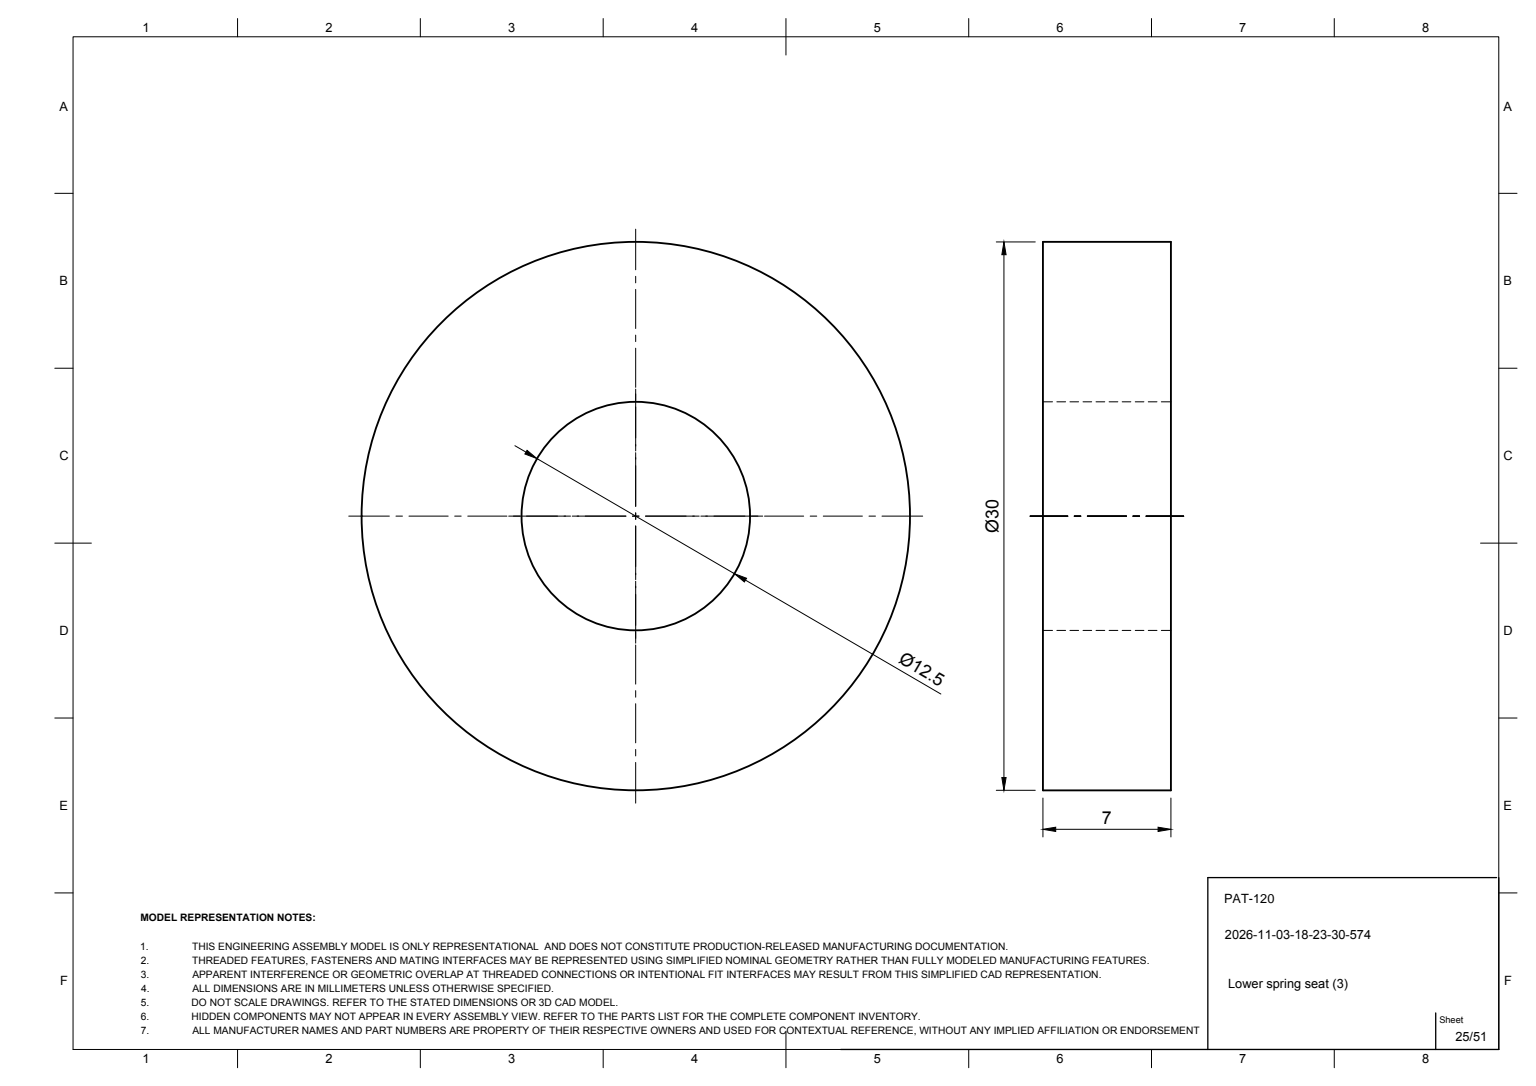
ISO-10303-21;
HEADER;
/* Generated by software containing ST-Developer
 * from STEP Tools, Inc. (www.steptools.com) 
 */

FILE_DESCRIPTION(
/* description */ ('Vibration shaker table dummy'),
/* implementation_level */ '2;1');

FILE_NAME(
/* name */ 'Lower spring seat (3).step',
/* time_stamp */ '2026-10-27T10:55:14-07:00',
/* author */ (''),
/* organization */ (''),
/* preprocessor_version */ 'ST-DEVELOPER v20.2',
/* originating_system */ 'Autodesk Translation Framework v15.17.0.0',
/* authorisation */ '');

FILE_SCHEMA (('AUTOMOTIVE_DESIGN { 1 0 10303 214 3 1 1 }'));
ENDSEC;

DATA;
#10=MECHANICAL_DESIGN_GEOMETRIC_PRESENTATION_REPRESENTATION('',(#706),#22394);
#614=SHAPE_REPRESENTATION_RELATIONSHIP('SRR','None',#22660,#660);
#660=ADVANCED_BREP_SHAPE_REPRESENTATION('',(#752),#22366);
#706=STYLED_ITEM('',(#22961),#752);
#752=MANIFOLD_SOLID_BREP('Body1',#9224);
#917=FACE_BOUND('',#2201,.T.);
#918=FACE_BOUND('',#2203,.T.);
#1188=PLANE('',#10197);
#1189=PLANE('',#10198);
#1558=FACE_OUTER_BOUND('',#2198,.T.);
#1559=FACE_OUTER_BOUND('',#2199,.T.);
#1560=FACE_OUTER_BOUND('',#2200,.T.);
#1561=FACE_OUTER_BOUND('',#2202,.T.);
#2198=EDGE_LOOP('',(#7260,#7261,#7262,#7263));
#2199=EDGE_LOOP('',(#7264,#7265,#7266,#7267));
#2200=EDGE_LOOP('',(#7268));
#2201=EDGE_LOOP('',(#7269));
#2202=EDGE_LOOP('',(#7270));
#2203=EDGE_LOOP('',(#7271));
#2932=LINE('',#19421,#3551);
#2933=LINE('',#19427,#3552);
#3551=VECTOR('',#12126,0.625);
#3552=VECTOR('',#12133,1.5);
#4054=CIRCLE('',#10192,0.625);
#4055=CIRCLE('',#10193,0.625);
#4056=CIRCLE('',#10195,1.5);
#4057=CIRCLE('',#10196,1.5);
#4705=VERTEX_POINT('',#19418);
#4706=VERTEX_POINT('',#19420);
#4707=VERTEX_POINT('',#19424);
#4708=VERTEX_POINT('',#19426);
#5623=EDGE_CURVE('',#4705,#4705,#4054,.T.);
#5624=EDGE_CURVE('',#4705,#4706,#2932,.T.);
#5625=EDGE_CURVE('',#4706,#4706,#4055,.T.);
#5626=EDGE_CURVE('',#4707,#4707,#4056,.T.);
#5627=EDGE_CURVE('',#4707,#4708,#2933,.T.);
#5628=EDGE_CURVE('',#4708,#4708,#4057,.T.);
#7260=ORIENTED_EDGE('',*,*,#5623,.F.);
#7261=ORIENTED_EDGE('',*,*,#5624,.T.);
#7262=ORIENTED_EDGE('',*,*,#5625,.T.);
#7263=ORIENTED_EDGE('',*,*,#5624,.F.);
#7264=ORIENTED_EDGE('',*,*,#5626,.F.);
#7265=ORIENTED_EDGE('',*,*,#5627,.T.);
#7266=ORIENTED_EDGE('',*,*,#5628,.T.);
#7267=ORIENTED_EDGE('',*,*,#5627,.F.);
#7268=ORIENTED_EDGE('',*,*,#5626,.T.);
#7269=ORIENTED_EDGE('',*,*,#5623,.T.);
#7270=ORIENTED_EDGE('',*,*,#5628,.F.);
#7271=ORIENTED_EDGE('',*,*,#5625,.F.);
#8592=CYLINDRICAL_SURFACE('',#10191,0.625);
#8593=CYLINDRICAL_SURFACE('',#10194,1.5);
#8923=ADVANCED_FACE('',(#1558),#8592,.F.);
#8924=ADVANCED_FACE('',(#1559),#8593,.T.);
#8925=ADVANCED_FACE('',(#1560,#917),#1188,.T.);
#8926=ADVANCED_FACE('',(#1561,#918),#1189,.F.);
#9224=CLOSED_SHELL('',(#8923,#8924,#8925,#8926));
#10190=AXIS2_PLACEMENT_3D('',#19416,#12120,#12121);
#10191=AXIS2_PLACEMENT_3D('',#19417,#12122,#12123);
#10192=AXIS2_PLACEMENT_3D('',#19419,#12124,#12125);
#10193=AXIS2_PLACEMENT_3D('',#19422,#12127,#12128);
#10194=AXIS2_PLACEMENT_3D('',#19423,#12129,#12130);
#10195=AXIS2_PLACEMENT_3D('',#19425,#12131,#12132);
#10196=AXIS2_PLACEMENT_3D('',#19428,#12134,#12135);
#10197=AXIS2_PLACEMENT_3D('',#19429,#12136,#12137);
#10198=AXIS2_PLACEMENT_3D('',#19430,#12138,#12139);
#12120=DIRECTION('axis',(0.,0.,1.));
#12121=DIRECTION('refdir',(1.,0.,0.));
#12122=DIRECTION('center_axis',(0.,0.,1.));
#12123=DIRECTION('ref_axis',(1.,0.,0.));
#12124=DIRECTION('center_axis',(0.,0.,-1.));
#12125=DIRECTION('ref_axis',(1.,0.,0.));
#12126=DIRECTION('',(0.,0.,-1.));
#12127=DIRECTION('center_axis',(0.,0.,-1.));
#12128=DIRECTION('ref_axis',(1.,0.,0.));
#12129=DIRECTION('center_axis',(0.,0.,1.));
#12130=DIRECTION('ref_axis',(1.,0.,0.));
#12131=DIRECTION('center_axis',(0.,0.,1.));
#12132=DIRECTION('ref_axis',(1.,0.,0.));
#12133=DIRECTION('',(0.,0.,-1.));
#12134=DIRECTION('center_axis',(0.,0.,1.));
#12135=DIRECTION('ref_axis',(1.,0.,0.));
#12136=DIRECTION('center_axis',(0.,0.,1.));
#12137=DIRECTION('ref_axis',(1.,0.,0.));
#12138=DIRECTION('center_axis',(0.,0.,1.));
#12139=DIRECTION('ref_axis',(1.,0.,0.));
#19416=CARTESIAN_POINT('',(0.,0.,0.));
#19417=CARTESIAN_POINT('Origin',(6.,4.,1.9));
#19418=CARTESIAN_POINT('',(5.375,4.,2.6));
#19419=CARTESIAN_POINT('Origin',(6.,4.,2.6));
#19420=CARTESIAN_POINT('',(5.375,4.,1.9));
#19421=CARTESIAN_POINT('',(5.375,4.,1.9));
#19422=CARTESIAN_POINT('Origin',(6.,4.,1.9));
#19423=CARTESIAN_POINT('Origin',(6.,4.,1.9));
#19424=CARTESIAN_POINT('',(4.5,4.,2.6));
#19425=CARTESIAN_POINT('Origin',(6.,4.,2.6));
#19426=CARTESIAN_POINT('',(4.5,4.,1.9));
#19427=CARTESIAN_POINT('',(4.5,4.,1.9));
#19428=CARTESIAN_POINT('Origin',(6.,4.,1.9));
#19429=CARTESIAN_POINT('Origin',(6.,4.,2.6));
#19430=CARTESIAN_POINT('Origin',(6.,4.,1.9));
#22315=UNCERTAINTY_MEASURE_WITH_UNIT(LENGTH_MEASURE(0.001),#22395,
'DISTANCE_ACCURACY_VALUE',
'Maximum model space distance between geometric entities at asserted c
onnectivities');
#22343=UNCERTAINTY_MEASURE_WITH_UNIT(LENGTH_MEASURE(0.001),#22395,
'DISTANCE_ACCURACY_VALUE',
'Maximum model space distance between geometric entities at asserted c
onnectivities');
#22366=(
GEOMETRIC_REPRESENTATION_CONTEXT(3)
GLOBAL_UNCERTAINTY_ASSIGNED_CONTEXT((#22315))
GLOBAL_UNIT_ASSIGNED_CONTEXT((#22395,#22397,#22398))
REPRESENTATION_CONTEXT('','3D')
);
#22394=(
GEOMETRIC_REPRESENTATION_CONTEXT(3)
GLOBAL_UNCERTAINTY_ASSIGNED_CONTEXT((#22343))
GLOBAL_UNIT_ASSIGNED_CONTEXT((#22395,#22397,#22398))
REPRESENTATION_CONTEXT('','3D')
);
#22395=(
LENGTH_UNIT()
NAMED_UNIT(*)
SI_UNIT(.CENTI.,.METRE.)
);
#22397=(
NAMED_UNIT(*)
PLANE_ANGLE_UNIT()
SI_UNIT($,.RADIAN.)
);
#22398=(
NAMED_UNIT(*)
SI_UNIT($,.STERADIAN.)
SOLID_ANGLE_UNIT()
);
#22421=SHAPE_DEFINITION_REPRESENTATION(#22471,#22660);
#22471=PRODUCT_DEFINITION_SHAPE('',$,#22711);
#22660=SHAPE_REPRESENTATION('',(#10190),#22366);
#22688=PRODUCT_DEFINITION_CONTEXT('part definition',#22840,'design');
#22711=PRODUCT_DEFINITION('Lower spring seat (3)','Lower spring seat (3)',
#22761,#22688);
#22761=PRODUCT_DEFINITION_FORMATION('',$,#22864);
#22840=APPLICATION_CONTEXT(
'Core Data for Automotive Mechanical Design Process');
#22841=PRODUCT_CONTEXT('part definition',#22840,'mechanical');
#22864=PRODUCT('Lower spring seat (3)','Lower spring seat (3)',
'Lower spring seat (3)',(#22841));
#22955=COLOUR_RGB('Grey',0.48,0.52,0.57);
#22956=FILL_AREA_STYLE_COLOUR('',#22955);
#22957=FILL_AREA_STYLE('',(#22956));
#22958=SURFACE_STYLE_FILL_AREA(#22957);
#22959=SURFACE_SIDE_STYLE('',(#22958));
#22960=SURFACE_STYLE_USAGE(.BOTH.,#22959);
#22961=PRESENTATION_STYLE_ASSIGNMENT((#22960));
ENDSEC;
END-ISO-10303-21;
